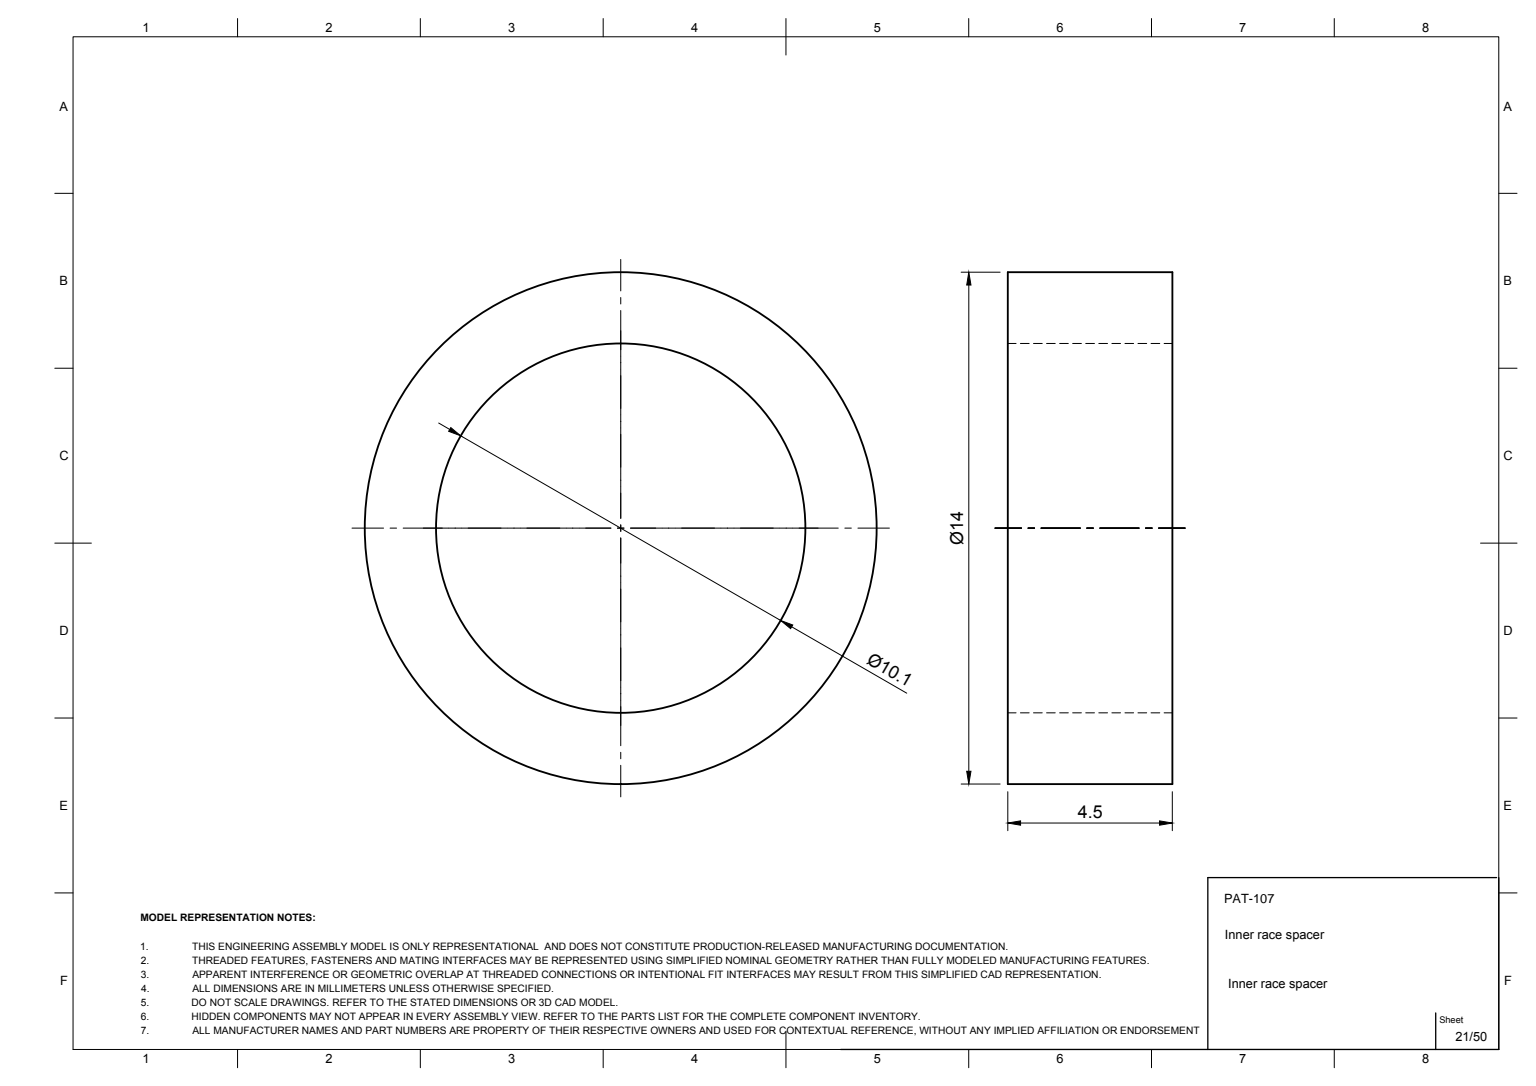
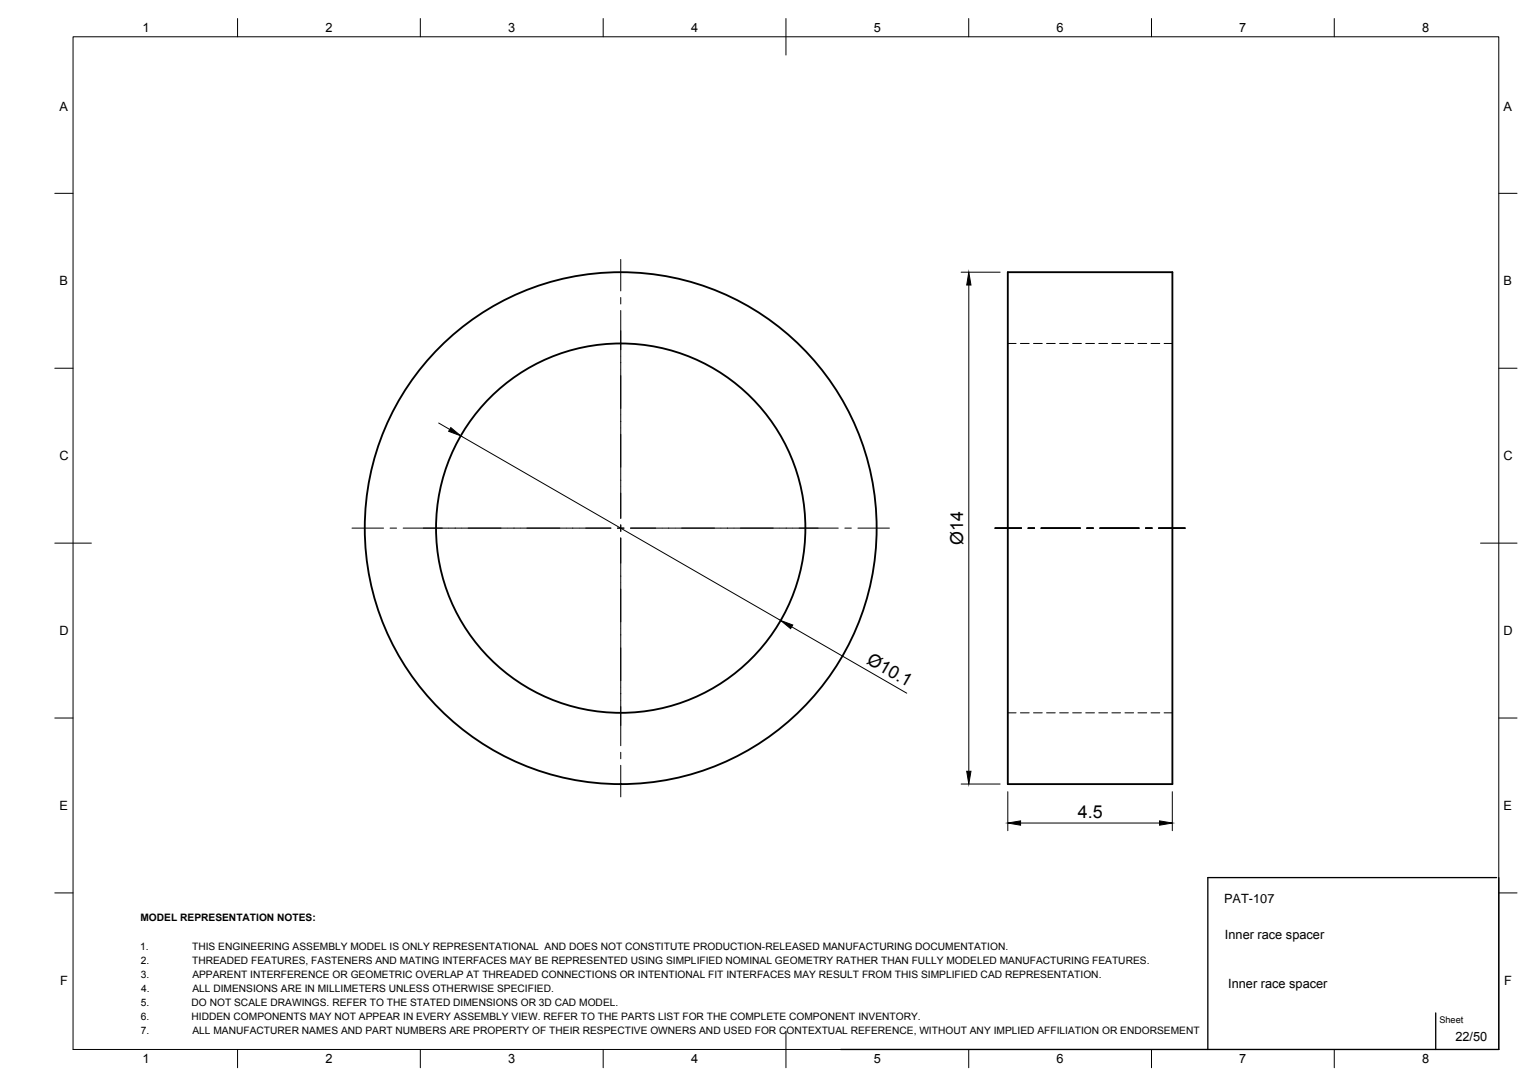
ISO-10303-21;
HEADER;
/* Generated by software containing ST-Developer
 * from STEP Tools, Inc. (www.steptools.com) 
 */

FILE_DESCRIPTION(
/* description */ ('Turntable on roller ring'),
/* implementation_level */ '2;1');

FILE_NAME(
/* name */ 'Inner race spacer.step',
/* time_stamp */ '2026-10-28T03:23:59-07:00',
/* author */ (''),
/* organization */ (''),
/* preprocessor_version */ 'ST-DEVELOPER v20.2',
/* originating_system */ 'Autodesk Translation Framework v15.17.0.0',
/* authorisation */ '');

FILE_SCHEMA (('AUTOMOTIVE_DESIGN { 1 0 10303 214 3 1 1 }'));
ENDSEC;

DATA;
#10=MECHANICAL_DESIGN_GEOMETRIC_PRESENTATION_REPRESENTATION('',(#644),#16281);
#525=SHAPE_REPRESENTATION_RELATIONSHIP('SRR','None',#16542,#580);
#580=ADVANCED_BREP_SHAPE_REPRESENTATION('',(#714),#16236);
#644=STYLED_ITEM('',(#16932),#714);
#714=MANIFOLD_SOLID_BREP('Body1',#8387);
#883=FACE_BOUND('',#2123,.T.);
#884=FACE_BOUND('',#2125,.T.);
#1103=PLANE('',#9589);
#1104=PLANE('',#9590);
#1489=FACE_OUTER_BOUND('',#2120,.T.);
#1490=FACE_OUTER_BOUND('',#2121,.T.);
#1491=FACE_OUTER_BOUND('',#2122,.T.);
#1492=FACE_OUTER_BOUND('',#2124,.T.);
#2120=EDGE_LOOP('',(#6671,#6672,#6673,#6674));
#2121=EDGE_LOOP('',(#6675,#6676,#6677,#6678));
#2122=EDGE_LOOP('',(#6679));
#2123=EDGE_LOOP('',(#6680));
#2124=EDGE_LOOP('',(#6681));
#2125=EDGE_LOOP('',(#6682));
#2731=LINE('',#14590,#3214);
#2732=LINE('',#14596,#3215);
#3214=VECTOR('',#11528,0.505);
#3215=VECTOR('',#11535,0.7);
#3713=CIRCLE('',#9584,0.505);
#3714=CIRCLE('',#9585,0.505);
#3715=CIRCLE('',#9587,0.7);
#3716=CIRCLE('',#9588,0.7);
#4293=VERTEX_POINT('',#14587);
#4294=VERTEX_POINT('',#14589);
#4295=VERTEX_POINT('',#14593);
#4296=VERTEX_POINT('',#14595);
#5146=EDGE_CURVE('',#4293,#4293,#3713,.T.);
#5147=EDGE_CURVE('',#4293,#4294,#2731,.T.);
#5148=EDGE_CURVE('',#4294,#4294,#3714,.T.);
#5149=EDGE_CURVE('',#4295,#4295,#3715,.T.);
#5150=EDGE_CURVE('',#4295,#4296,#2732,.T.);
#5151=EDGE_CURVE('',#4296,#4296,#3716,.T.);
#6671=ORIENTED_EDGE('',*,*,#5146,.F.);
#6672=ORIENTED_EDGE('',*,*,#5147,.T.);
#6673=ORIENTED_EDGE('',*,*,#5148,.T.);
#6674=ORIENTED_EDGE('',*,*,#5147,.F.);
#6675=ORIENTED_EDGE('',*,*,#5149,.F.);
#6676=ORIENTED_EDGE('',*,*,#5150,.T.);
#6677=ORIENTED_EDGE('',*,*,#5151,.T.);
#6678=ORIENTED_EDGE('',*,*,#5150,.F.);
#6679=ORIENTED_EDGE('',*,*,#5149,.T.);
#6680=ORIENTED_EDGE('',*,*,#5146,.T.);
#6681=ORIENTED_EDGE('',*,*,#5151,.F.);
#6682=ORIENTED_EDGE('',*,*,#5148,.F.);
#7762=CYLINDRICAL_SURFACE('',#9583,0.505);
#7763=CYLINDRICAL_SURFACE('',#9586,0.7);
#8092=ADVANCED_FACE('',(#1489),#7762,.F.);
#8093=ADVANCED_FACE('',(#1490),#7763,.T.);
#8094=ADVANCED_FACE('',(#1491,#883),#1103,.T.);
#8095=ADVANCED_FACE('',(#1492,#884),#1104,.F.);
#8387=CLOSED_SHELL('',(#8092,#8093,#8094,#8095));
#9582=AXIS2_PLACEMENT_3D('',#14585,#11522,#11523);
#9583=AXIS2_PLACEMENT_3D('',#14586,#11524,#11525);
#9584=AXIS2_PLACEMENT_3D('',#14588,#11526,#11527);
#9585=AXIS2_PLACEMENT_3D('',#14591,#11529,#11530);
#9586=AXIS2_PLACEMENT_3D('',#14592,#11531,#11532);
#9587=AXIS2_PLACEMENT_3D('',#14594,#11533,#11534);
#9588=AXIS2_PLACEMENT_3D('',#14597,#11536,#11537);
#9589=AXIS2_PLACEMENT_3D('',#14598,#11538,#11539);
#9590=AXIS2_PLACEMENT_3D('',#14599,#11540,#11541);
#11522=DIRECTION('axis',(0.,0.,1.));
#11523=DIRECTION('refdir',(1.,0.,0.));
#11524=DIRECTION('center_axis',(0.,1.,0.));
#11525=DIRECTION('ref_axis',(1.,0.,0.));
#11526=DIRECTION('center_axis',(0.,-1.,0.));
#11527=DIRECTION('ref_axis',(1.,0.,0.));
#11528=DIRECTION('',(0.,-1.,0.));
#11529=DIRECTION('center_axis',(0.,-1.,0.));
#11530=DIRECTION('ref_axis',(1.,0.,0.));
#11531=DIRECTION('center_axis',(0.,1.,0.));
#11532=DIRECTION('ref_axis',(1.,0.,0.));
#11533=DIRECTION('center_axis',(0.,1.,0.));
#11534=DIRECTION('ref_axis',(1.,0.,0.));
#11535=DIRECTION('',(0.,-1.,0.));
#11536=DIRECTION('center_axis',(0.,1.,0.));
#11537=DIRECTION('ref_axis',(1.,0.,0.));
#11538=DIRECTION('center_axis',(0.,1.,0.));
#11539=DIRECTION('ref_axis',(1.,0.,0.));
#11540=DIRECTION('center_axis',(0.,1.,0.));
#11541=DIRECTION('ref_axis',(1.,0.,0.));
#14585=CARTESIAN_POINT('',(0.,0.,0.));
#14586=CARTESIAN_POINT('Origin',(0.,14.1,3.5));
#14587=CARTESIAN_POINT('',(-0.505,14.55,3.5));
#14588=CARTESIAN_POINT('Origin',(0.,14.55,3.5));
#14589=CARTESIAN_POINT('',(-0.505,14.1,3.5));
#14590=CARTESIAN_POINT('',(-0.505,14.1,3.5));
#14591=CARTESIAN_POINT('Origin',(0.,14.1,3.5));
#14592=CARTESIAN_POINT('Origin',(0.,14.1,3.5));
#14593=CARTESIAN_POINT('',(-0.7,14.55,3.5));
#14594=CARTESIAN_POINT('Origin',(0.,14.55,3.5));
#14595=CARTESIAN_POINT('',(-0.7,14.1,3.5));
#14596=CARTESIAN_POINT('',(-0.7,14.1,3.5));
#14597=CARTESIAN_POINT('Origin',(0.,14.1,3.5));
#14598=CARTESIAN_POINT('Origin',(0.,14.55,3.5));
#14599=CARTESIAN_POINT('Origin',(0.,14.1,3.5));
#16167=UNCERTAINTY_MEASURE_WITH_UNIT(LENGTH_MEASURE(0.001),#16282,
'DISTANCE_ACCURACY_VALUE',
'Maximum model space distance between geometric entities at asserted c
onnectivities');
#16212=UNCERTAINTY_MEASURE_WITH_UNIT(LENGTH_MEASURE(0.001),#16282,
'DISTANCE_ACCURACY_VALUE',
'Maximum model space distance between geometric entities at asserted c
onnectivities');
#16236=(
GEOMETRIC_REPRESENTATION_CONTEXT(3)
GLOBAL_UNCERTAINTY_ASSIGNED_CONTEXT((#16167))
GLOBAL_UNIT_ASSIGNED_CONTEXT((#16282,#16284,#16285))
REPRESENTATION_CONTEXT('','3D')
);
#16281=(
GEOMETRIC_REPRESENTATION_CONTEXT(3)
GLOBAL_UNCERTAINTY_ASSIGNED_CONTEXT((#16212))
GLOBAL_UNIT_ASSIGNED_CONTEXT((#16282,#16284,#16285))
REPRESENTATION_CONTEXT('','3D')
);
#16282=(
LENGTH_UNIT()
NAMED_UNIT(*)
SI_UNIT(.CENTI.,.METRE.)
);
#16284=(
NAMED_UNIT(*)
PLANE_ANGLE_UNIT()
SI_UNIT($,.RADIAN.)
);
#16285=(
NAMED_UNIT(*)
SI_UNIT($,.STERADIAN.)
SOLID_ANGLE_UNIT()
);
#16309=SHAPE_DEFINITION_REPRESENTATION(#16403,#16542);
#16403=PRODUCT_DEFINITION_SHAPE('',$,#16611);
#16542=SHAPE_REPRESENTATION('',(#9582),#16236);
#16587=PRODUCT_DEFINITION_CONTEXT('part definition',#16793,'design');
#16611=PRODUCT_DEFINITION('Inner race spacer','Inner race spacer',#16679,
#16587);
#16679=PRODUCT_DEFINITION_FORMATION('',$,#16818);
#16793=APPLICATION_CONTEXT(
'Core Data for Automotive Mechanical Design Process');
#16794=PRODUCT_CONTEXT('part definition',#16793,'mechanical');
#16818=PRODUCT('Inner race spacer','Inner race spacer',
'Inner race spacer',(#16794));
#16926=COLOUR_RGB('Grey',0.48,0.52,0.57);
#16927=FILL_AREA_STYLE_COLOUR('',#16926);
#16928=FILL_AREA_STYLE('',(#16927));
#16929=SURFACE_STYLE_FILL_AREA(#16928);
#16930=SURFACE_SIDE_STYLE('',(#16929));
#16931=SURFACE_STYLE_USAGE(.BOTH.,#16930);
#16932=PRESENTATION_STYLE_ASSIGNMENT((#16931));
ENDSEC;
END-ISO-10303-21;
